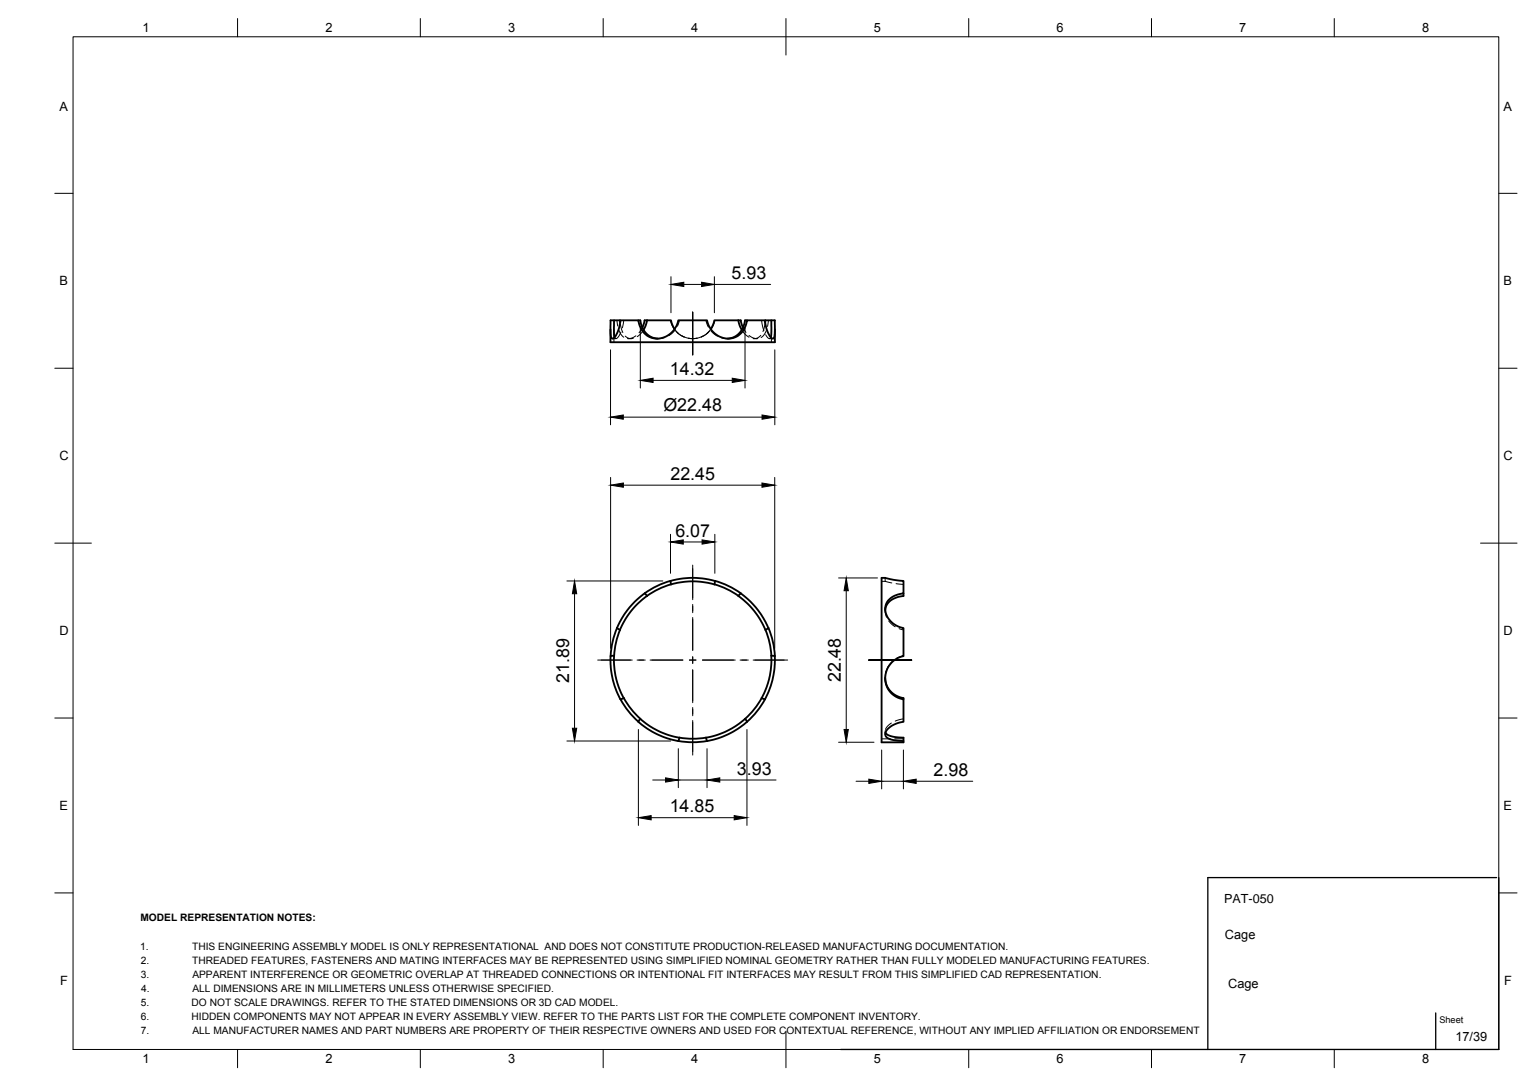
ISO-10303-21;
HEADER;
/* Generated by software containing ST-Developer
 * from STEP Tools, Inc. (www.steptools.com) 
 */

FILE_DESCRIPTION(
/* description */ ('Hand wheel with handle and shaft collar'),
/* implementation_level */ '2;1');

FILE_NAME(
/* name */ 'Cage.step',
/* time_stamp */ '2026-10-28T03:23:19-07:00',
/* author */ (''),
/* organization */ (''),
/* preprocessor_version */ 'ST-DEVELOPER v20.2',
/* originating_system */ 'Autodesk Translation Framework v15.17.0.0',
/* authorisation */ '');

FILE_SCHEMA (('AUTOMOTIVE_DESIGN { 1 0 10303 214 3 1 1 }'));
ENDSEC;

DATA;
#10=MECHANICAL_DESIGN_GEOMETRIC_PRESENTATION_REPRESENTATION('',(#413),#10510);
#227=B_SPLINE_CURVE_WITH_KNOTS('',3,(#8677,#8678,#8679,#8680,#8681,#8682,
#8683,#8684,#8685,#8686,#8687,#8688,#8689,#8690,#8691,#8692,#8693,#8694,
#8695,#8696,#8697,#8698),.UNSPECIFIED.,.F.,.F.,(4,2,2,2,2,2,2,2,2,2,4),
(0.0591825211272536,0.157966726598481,0.236950089897721,0.315933453196962,
0.391576304923761,0.46721915665056,0.54286200837736,0.618504860104159,0.697488223403399,
0.77647158670264,0.875255792173867),.UNSPECIFIED.);
#228=B_SPLINE_CURVE_WITH_KNOTS('',3,(#8702,#8703,#8704,#8705,#8706,#8707,
#8708,#8709,#8710,#8711,#8712,#8713,#8714,#8715,#8716,#8717,#8718,#8719,
#8720,#8721,#8722,#8723),.UNSPECIFIED.,.F.,.F.,(4,2,2,2,2,2,2,2,2,2,4),
(0.0581119756758434,0.106553146291161,0.213106292582322,0.30849933801665,
0.386091982889075,0.4636846277615,0.541277272633925,0.61886991750635,0.714262962940678,
0.820816109231839,0.869257279847157),.UNSPECIFIED.);
#229=B_SPLINE_CURVE_WITH_KNOTS('',3,(#8729,#8730,#8731,#8732,#8733,#8734,
#8735,#8736,#8737,#8738,#8739,#8740,#8741,#8742,#8743,#8744,#8745,#8746,
#8747,#8748,#8749,#8750),.UNSPECIFIED.,.F.,.F.,(4,2,2,2,2,2,2,2,2,2,4),
(0.0581119756758434,0.106553146291161,0.213106292582322,0.30849933801665,
0.386091982889075,0.4636846277615,0.541277272633925,0.61886991750635,0.714262962940679,
0.820816109231839,0.869257279847157),.UNSPECIFIED.);
#230=B_SPLINE_CURVE_WITH_KNOTS('',3,(#8754,#8755,#8756,#8757,#8758,#8759,
#8760,#8761,#8762,#8763,#8764,#8765,#8766,#8767,#8768,#8769,#8770,#8771,
#8772,#8773,#8774,#8775),.UNSPECIFIED.,.F.,.F.,(4,2,2,2,2,2,2,2,2,2,4),
(0.0581119756758433,0.106553146291161,0.213106292582322,0.308499338016649,
0.386091982889075,0.4636846277615,0.541277272633925,0.61886991750635,0.714262962940678,
0.820816109231839,0.869257279847157),.UNSPECIFIED.);
#231=B_SPLINE_CURVE_WITH_KNOTS('',3,(#8784,#8785,#8786,#8787,#8788,#8789,
#8790,#8791,#8792,#8793,#8794,#8795,#8796,#8797,#8798,#8799,#8800,#8801,
#8802,#8803,#8804,#8805),.UNSPECIFIED.,.F.,.F.,(4,2,2,2,2,2,2,2,2,2,4),
(0.0581119756758433,0.106553146291161,0.213106292582322,0.30849933801665,
0.386091982889075,0.4636846277615,0.541277272633925,0.61886991750635,0.714262962940678,
0.820816109231839,0.869257279847157),.UNSPECIFIED.);
#232=B_SPLINE_CURVE_WITH_KNOTS('',3,(#8809,#8810,#8811,#8812,#8813,#8814,
#8815,#8816,#8817,#8818,#8819,#8820,#8821,#8822,#8823,#8824,#8825,#8826,
#8827,#8828,#8829,#8830),.UNSPECIFIED.,.F.,.F.,(4,2,2,2,2,2,2,2,2,2,4),
(0.0581119756758434,0.106553146291161,0.213106292582322,0.30849933801665,
0.386091982889075,0.4636846277615,0.541277272633925,0.61886991750635,0.714262962940678,
0.820816109231839,0.869257279847157),.UNSPECIFIED.);
#233=B_SPLINE_CURVE_WITH_KNOTS('',3,(#8834,#8835,#8836,#8837,#8838,#8839,
#8840,#8841,#8842,#8843,#8844,#8845,#8846,#8847,#8848,#8849,#8850,#8851,
#8852,#8853,#8854,#8855),.UNSPECIFIED.,.F.,.F.,(4,2,2,2,2,2,2,2,2,2,4),
(0.0581119756758434,0.106553146291161,0.213106292582322,0.30849933801665,
0.386091982889075,0.4636846277615,0.541277272633925,0.61886991750635,0.714262962940678,
0.820816109231839,0.869257279847157),.UNSPECIFIED.);
#234=B_SPLINE_CURVE_WITH_KNOTS('',3,(#8859,#8860,#8861,#8862,#8863,#8864,
#8865,#8866,#8867,#8868,#8869,#8870,#8871,#8872,#8873,#8874,#8875,#8876,
#8877,#8878,#8879,#8880),.UNSPECIFIED.,.F.,.F.,(4,2,2,2,2,2,2,2,2,2,4),
(0.0581119756758433,0.106553146291161,0.213106292582322,0.30849933801665,
0.386091982889075,0.4636846277615,0.541277272633925,0.61886991750635,0.714262962940678,
0.820816109231839,0.869257279847157),.UNSPECIFIED.);
#235=B_SPLINE_CURVE_WITH_KNOTS('',3,(#8888,#8889,#8890,#8891,#8892,#8893,
#8894,#8895,#8896,#8897,#8898,#8899,#8900,#8901,#8902,#8903,#8904,#8905,
#8906,#8907,#8908,#8909),.UNSPECIFIED.,.F.,.F.,(4,2,2,2,2,2,2,2,2,2,4),
(0.0591825211272536,0.157966726598481,0.236950089897721,0.315933453196962,
0.391576304923761,0.467219156650561,0.54286200837736,0.618504860104159,
0.697488223403399,0.77647158670264,0.875255792173867),.UNSPECIFIED.);
#236=B_SPLINE_CURVE_WITH_KNOTS('',3,(#8917,#8918,#8919,#8920,#8921,#8922,
#8923,#8924,#8925,#8926,#8927,#8928,#8929,#8930,#8931,#8932,#8933,#8934,
#8935,#8936,#8937,#8938),.UNSPECIFIED.,.F.,.F.,(4,2,2,2,2,2,2,2,2,2,4),
(0.0591825211272536,0.157966726598481,0.236950089897722,0.315933453196962,
0.391576304923761,0.467219156650561,0.54286200837736,0.618504860104159,
0.697488223403399,0.77647158670264,0.875255792173867),.UNSPECIFIED.);
#237=B_SPLINE_CURVE_WITH_KNOTS('',3,(#8948,#8949,#8950,#8951,#8952,#8953,
#8954,#8955,#8956,#8957,#8958,#8959,#8960,#8961,#8962,#8963,#8964,#8965,
#8966,#8967,#8968,#8969),.UNSPECIFIED.,.F.,.F.,(4,2,2,2,2,2,2,2,2,2,4),
(0.0591825211272536,0.157966726598481,0.236950089897721,0.315933453196962,
0.391576304923761,0.46721915665056,0.54286200837736,0.618504860104159,0.697488223403399,
0.77647158670264,0.875255792173867),.UNSPECIFIED.);
#238=B_SPLINE_CURVE_WITH_KNOTS('',3,(#8977,#8978,#8979,#8980,#8981,#8982,
#8983,#8984,#8985,#8986,#8987,#8988,#8989,#8990,#8991,#8992,#8993,#8994,
#8995,#8996,#8997,#8998),.UNSPECIFIED.,.F.,.F.,(4,2,2,2,2,2,2,2,2,2,4),
(0.0591825211272536,0.157966726598481,0.236950089897721,0.315933453196962,
0.391576304923761,0.46721915665056,0.542862008377359,0.618504860104159,
0.697488223403399,0.776471586702639,0.875255792173867),.UNSPECIFIED.);
#239=B_SPLINE_CURVE_WITH_KNOTS('',3,(#9006,#9007,#9008,#9009,#9010,#9011,
#9012,#9013,#9014,#9015,#9016,#9017,#9018,#9019,#9020,#9021,#9022,#9023,
#9024,#9025,#9026,#9027),.UNSPECIFIED.,.F.,.F.,(4,2,2,2,2,2,2,2,2,2,4),
(0.0591825211272536,0.157966726598481,0.236950089897721,0.315933453196962,
0.391576304923761,0.46721915665056,0.54286200837736,0.618504860104159,0.697488223403399,
0.77647158670264,0.875255792173867),.UNSPECIFIED.);
#240=B_SPLINE_CURVE_WITH_KNOTS('',3,(#9036,#9037,#9038,#9039,#9040,#9041,
#9042,#9043,#9044,#9045,#9046,#9047,#9048,#9049,#9050,#9051,#9052,#9053,
#9054,#9055,#9056,#9057),.UNSPECIFIED.,.F.,.F.,(4,2,2,2,2,2,2,2,2,2,4),
(0.0591825211272536,0.157966726598481,0.236950089897721,0.315933453196962,
0.391576304923761,0.46721915665056,0.542862008377359,0.618504860104159,
0.697488223403399,0.776471586702639,0.875255792173867),.UNSPECIFIED.);
#274=SPHERICAL_SURFACE('',#5919,0.309556);
#275=SPHERICAL_SURFACE('',#5935,0.309556);
#276=SPHERICAL_SURFACE('',#5940,0.309556);
#277=SPHERICAL_SURFACE('',#5946,0.309556);
#278=SPHERICAL_SURFACE('',#5951,0.309556);
#279=SPHERICAL_SURFACE('',#5956,0.309556);
#280=SPHERICAL_SURFACE('',#5964,0.309556);
#343=SHAPE_REPRESENTATION_RELATIONSHIP('SRR','None',#10660,#375);
#375=ADVANCED_BREP_SHAPE_REPRESENTATION('',(#459),#10487);
#413=STYLED_ITEM('',(#10908),#459);
#459=MANIFOLD_SOLID_BREP('Continuous crown cage',#5313);
#543=FACE_BOUND('',#1263,.T.);
#651=PLANE('',#5932);
#652=PLANE('',#5937);
#653=PLANE('',#5942);
#654=PLANE('',#5948);
#655=PLANE('',#5953);
#656=PLANE('',#5962);
#657=PLANE('',#5966);
#658=PLANE('',#5967);
#871=FACE_OUTER_BOUND('',#1247,.T.);
#872=FACE_OUTER_BOUND('',#1248,.T.);
#873=FACE_OUTER_BOUND('',#1249,.T.);
#874=FACE_OUTER_BOUND('',#1250,.T.);
#875=FACE_OUTER_BOUND('',#1251,.T.);
#876=FACE_OUTER_BOUND('',#1252,.T.);
#877=FACE_OUTER_BOUND('',#1253,.T.);
#878=FACE_OUTER_BOUND('',#1254,.T.);
#879=FACE_OUTER_BOUND('',#1255,.T.);
#880=FACE_OUTER_BOUND('',#1256,.T.);
#881=FACE_OUTER_BOUND('',#1257,.T.);
#882=FACE_OUTER_BOUND('',#1258,.T.);
#883=FACE_OUTER_BOUND('',#1259,.T.);
#884=FACE_OUTER_BOUND('',#1260,.T.);
#885=FACE_OUTER_BOUND('',#1261,.T.);
#886=FACE_OUTER_BOUND('',#1262,.T.);
#887=FACE_OUTER_BOUND('',#1264,.T.);
#1247=EDGE_LOOP('',(#4001,#4002,#4003,#4004));
#1248=EDGE_LOOP('',(#4005,#4006,#4007,#4008,#4009,#4010,#4011,#4012,#4013,
#4014,#4015,#4016,#4017,#4018,#4019,#4020,#4021,#4022));
#1249=EDGE_LOOP('',(#4023,#4024,#4025,#4026));
#1250=EDGE_LOOP('',(#4027,#4028,#4029,#4030));
#1251=EDGE_LOOP('',(#4031,#4032,#4033,#4034));
#1252=EDGE_LOOP('',(#4035,#4036,#4037,#4038));
#1253=EDGE_LOOP('',(#4039,#4040,#4041,#4042,#4043,#4044));
#1254=EDGE_LOOP('',(#4045,#4046,#4047,#4048));
#1255=EDGE_LOOP('',(#4049,#4050,#4051,#4052));
#1256=EDGE_LOOP('',(#4053,#4054,#4055,#4056));
#1257=EDGE_LOOP('',(#4057,#4058,#4059,#4060));
#1258=EDGE_LOOP('',(#4061,#4062,#4063,#4064));
#1259=EDGE_LOOP('',(#4065,#4066,#4067,#4068,#4069,#4070,#4071,#4072,#4073,
#4074,#4075,#4076,#4077,#4078,#4079,#4080,#4081,#4082));
#1260=EDGE_LOOP('',(#4083,#4084,#4085,#4086));
#1261=EDGE_LOOP('',(#4087,#4088,#4089,#4090));
#1262=EDGE_LOOP('',(#4091));
#1263=EDGE_LOOP('',(#4092));
#1264=EDGE_LOOP('',(#4093,#4094,#4095,#4096));
#1637=LINE('',#8779,#1947);
#1638=LINE('',#9032,#1948);
#1947=VECTOR('',#7001,1.123812);
#1948=VECTOR('',#7070,1.076188);
#2231=CIRCLE('',#5920,0.303778037777585);
#2232=CIRCLE('',#5921,0.303778037777585);
#2233=CIRCLE('',#5923,1.123812);
#2234=CIRCLE('',#5924,1.123812);
#2235=CIRCLE('',#5925,1.123812);
#2236=CIRCLE('',#5926,1.123812);
#2237=CIRCLE('',#5927,1.123812);
#2238=CIRCLE('',#5928,1.123812);
#2239=CIRCLE('',#5929,1.123812);
#2240=CIRCLE('',#5930,1.123812);
#2241=CIRCLE('',#5931,1.123812);
#2242=CIRCLE('',#5933,1.076188);
#2243=CIRCLE('',#5934,0.303778037777585);
#2244=CIRCLE('',#5936,0.303778037777585);
#2245=CIRCLE('',#5938,1.076188);
#2246=CIRCLE('',#5939,0.303778037777585);
#2247=CIRCLE('',#5941,0.303778037777585);
#2248=CIRCLE('',#5943,1.076188);
#2249=CIRCLE('',#5944,1.076188);
#2250=CIRCLE('',#5945,0.303778037777585);
#2251=CIRCLE('',#5947,0.303778037777585);
#2252=CIRCLE('',#5949,1.076188);
#2253=CIRCLE('',#5950,0.303778037777585);
#2254=CIRCLE('',#5952,0.303778037777585);
#2255=CIRCLE('',#5954,1.076188);
#2256=CIRCLE('',#5955,0.303778037777585);
#2257=CIRCLE('',#5957,0.303778037777585);
#2258=CIRCLE('',#5959,1.076188);
#2259=CIRCLE('',#5960,1.076188);
#2260=CIRCLE('',#5961,1.076188);
#2261=CIRCLE('',#5963,0.303778037777585);
#2262=CIRCLE('',#5965,0.303778037777585);
#2599=VERTEX_POINT('',#8675);
#2600=VERTEX_POINT('',#8676);
#2601=VERTEX_POINT('',#8699);
#2602=VERTEX_POINT('',#8701);
#2603=VERTEX_POINT('',#8726);
#2604=VERTEX_POINT('',#8728);
#2605=VERTEX_POINT('',#8751);
#2606=VERTEX_POINT('',#8753);
#2607=VERTEX_POINT('',#8776);
#2608=VERTEX_POINT('',#8778);
#2609=VERTEX_POINT('',#8781);
#2610=VERTEX_POINT('',#8783);
#2611=VERTEX_POINT('',#8806);
#2612=VERTEX_POINT('',#8808);
#2613=VERTEX_POINT('',#8831);
#2614=VERTEX_POINT('',#8833);
#2615=VERTEX_POINT('',#8856);
#2616=VERTEX_POINT('',#8858);
#2617=VERTEX_POINT('',#8883);
#2618=VERTEX_POINT('',#8887);
#2619=VERTEX_POINT('',#8912);
#2620=VERTEX_POINT('',#8916);
#2621=VERTEX_POINT('',#8941);
#2622=VERTEX_POINT('',#8943);
#2623=VERTEX_POINT('',#8947);
#2624=VERTEX_POINT('',#8972);
#2625=VERTEX_POINT('',#8976);
#2626=VERTEX_POINT('',#9001);
#2627=VERTEX_POINT('',#9005);
#2628=VERTEX_POINT('',#9030);
#2629=VERTEX_POINT('',#9033);
#2630=VERTEX_POINT('',#9035);
#3118=EDGE_CURVE('',#2599,#2600,#227,.T.);
#3119=EDGE_CURVE('',#2601,#2599,#2231,.T.);
#3120=EDGE_CURVE('',#2602,#2601,#228,.T.);
#3121=EDGE_CURVE('',#2600,#2602,#2232,.T.);
#3122=EDGE_CURVE('',#2603,#2601,#2233,.T.);
#3123=EDGE_CURVE('',#2603,#2604,#229,.T.);
#3124=EDGE_CURVE('',#2605,#2604,#2234,.T.);
#3125=EDGE_CURVE('',#2605,#2606,#230,.T.);
#3126=EDGE_CURVE('',#2607,#2606,#2235,.T.);
#3127=EDGE_CURVE('',#2607,#2608,#1637,.T.);
#3128=EDGE_CURVE('',#2608,#2608,#2236,.T.);
#3129=EDGE_CURVE('',#2609,#2607,#2237,.T.);
#3130=EDGE_CURVE('',#2609,#2610,#231,.T.);
#3131=EDGE_CURVE('',#2611,#2610,#2238,.T.);
#3132=EDGE_CURVE('',#2611,#2612,#232,.T.);
#3133=EDGE_CURVE('',#2613,#2612,#2239,.T.);
#3134=EDGE_CURVE('',#2613,#2614,#233,.T.);
#3135=EDGE_CURVE('',#2615,#2614,#2240,.T.);
#3136=EDGE_CURVE('',#2615,#2616,#234,.T.);
#3137=EDGE_CURVE('',#2602,#2616,#2241,.T.);
#3138=EDGE_CURVE('',#2599,#2617,#2242,.T.);
#3139=EDGE_CURVE('',#2617,#2603,#2243,.T.);
#3140=EDGE_CURVE('',#2618,#2617,#235,.T.);
#3141=EDGE_CURVE('',#2604,#2618,#2244,.T.);
#3142=EDGE_CURVE('',#2618,#2619,#2245,.T.);
#3143=EDGE_CURVE('',#2619,#2605,#2246,.T.);
#3144=EDGE_CURVE('',#2620,#2619,#236,.T.);
#3145=EDGE_CURVE('',#2606,#2620,#2247,.T.);
#3146=EDGE_CURVE('',#2620,#2621,#2248,.T.);
#3147=EDGE_CURVE('',#2621,#2622,#2249,.T.);
#3148=EDGE_CURVE('',#2622,#2609,#2250,.T.);
#3149=EDGE_CURVE('',#2623,#2622,#237,.T.);
#3150=EDGE_CURVE('',#2610,#2623,#2251,.T.);
#3151=EDGE_CURVE('',#2623,#2624,#2252,.T.);
#3152=EDGE_CURVE('',#2624,#2611,#2253,.T.);
#3153=EDGE_CURVE('',#2625,#2624,#238,.T.);
#3154=EDGE_CURVE('',#2612,#2625,#2254,.T.);
#3155=EDGE_CURVE('',#2625,#2626,#2255,.T.);
#3156=EDGE_CURVE('',#2626,#2613,#2256,.T.);
#3157=EDGE_CURVE('',#2627,#2626,#239,.T.);
#3158=EDGE_CURVE('',#2614,#2627,#2257,.T.);
#3159=EDGE_CURVE('',#2628,#2628,#2258,.T.);
#3160=EDGE_CURVE('',#2628,#2621,#1638,.T.);
#3161=EDGE_CURVE('',#2629,#2600,#2259,.T.);
#3162=EDGE_CURVE('',#2629,#2630,#240,.T.);
#3163=EDGE_CURVE('',#2627,#2630,#2260,.T.);
#3164=EDGE_CURVE('',#2616,#2629,#2261,.T.);
#3165=EDGE_CURVE('',#2630,#2615,#2262,.T.);
#4001=ORIENTED_EDGE('',*,*,#3118,.F.);
#4002=ORIENTED_EDGE('',*,*,#3119,.F.);
#4003=ORIENTED_EDGE('',*,*,#3120,.F.);
#4004=ORIENTED_EDGE('',*,*,#3121,.F.);
#4005=ORIENTED_EDGE('',*,*,#3120,.T.);
#4006=ORIENTED_EDGE('',*,*,#3122,.F.);
#4007=ORIENTED_EDGE('',*,*,#3123,.T.);
#4008=ORIENTED_EDGE('',*,*,#3124,.F.);
#4009=ORIENTED_EDGE('',*,*,#3125,.T.);
#4010=ORIENTED_EDGE('',*,*,#3126,.F.);
#4011=ORIENTED_EDGE('',*,*,#3127,.T.);
#4012=ORIENTED_EDGE('',*,*,#3128,.F.);
#4013=ORIENTED_EDGE('',*,*,#3127,.F.);
#4014=ORIENTED_EDGE('',*,*,#3129,.F.);
#4015=ORIENTED_EDGE('',*,*,#3130,.T.);
#4016=ORIENTED_EDGE('',*,*,#3131,.F.);
#4017=ORIENTED_EDGE('',*,*,#3132,.T.);
#4018=ORIENTED_EDGE('',*,*,#3133,.F.);
#4019=ORIENTED_EDGE('',*,*,#3134,.T.);
#4020=ORIENTED_EDGE('',*,*,#3135,.F.);
#4021=ORIENTED_EDGE('',*,*,#3136,.T.);
#4022=ORIENTED_EDGE('',*,*,#3137,.F.);
#4023=ORIENTED_EDGE('',*,*,#3119,.T.);
#4024=ORIENTED_EDGE('',*,*,#3138,.T.);
#4025=ORIENTED_EDGE('',*,*,#3139,.T.);
#4026=ORIENTED_EDGE('',*,*,#3122,.T.);
#4027=ORIENTED_EDGE('',*,*,#3140,.F.);
#4028=ORIENTED_EDGE('',*,*,#3141,.F.);
#4029=ORIENTED_EDGE('',*,*,#3123,.F.);
#4030=ORIENTED_EDGE('',*,*,#3139,.F.);
#4031=ORIENTED_EDGE('',*,*,#3141,.T.);
#4032=ORIENTED_EDGE('',*,*,#3142,.T.);
#4033=ORIENTED_EDGE('',*,*,#3143,.T.);
#4034=ORIENTED_EDGE('',*,*,#3124,.T.);
#4035=ORIENTED_EDGE('',*,*,#3144,.F.);
#4036=ORIENTED_EDGE('',*,*,#3145,.F.);
#4037=ORIENTED_EDGE('',*,*,#3125,.F.);
#4038=ORIENTED_EDGE('',*,*,#3143,.F.);
#4039=ORIENTED_EDGE('',*,*,#3145,.T.);
#4040=ORIENTED_EDGE('',*,*,#3146,.T.);
#4041=ORIENTED_EDGE('',*,*,#3147,.T.);
#4042=ORIENTED_EDGE('',*,*,#3148,.T.);
#4043=ORIENTED_EDGE('',*,*,#3129,.T.);
#4044=ORIENTED_EDGE('',*,*,#3126,.T.);
#4045=ORIENTED_EDGE('',*,*,#3149,.F.);
#4046=ORIENTED_EDGE('',*,*,#3150,.F.);
#4047=ORIENTED_EDGE('',*,*,#3130,.F.);
#4048=ORIENTED_EDGE('',*,*,#3148,.F.);
#4049=ORIENTED_EDGE('',*,*,#3150,.T.);
#4050=ORIENTED_EDGE('',*,*,#3151,.T.);
#4051=ORIENTED_EDGE('',*,*,#3152,.T.);
#4052=ORIENTED_EDGE('',*,*,#3131,.T.);
#4053=ORIENTED_EDGE('',*,*,#3153,.F.);
#4054=ORIENTED_EDGE('',*,*,#3154,.F.);
#4055=ORIENTED_EDGE('',*,*,#3132,.F.);
#4056=ORIENTED_EDGE('',*,*,#3152,.F.);
#4057=ORIENTED_EDGE('',*,*,#3154,.T.);
#4058=ORIENTED_EDGE('',*,*,#3155,.T.);
#4059=ORIENTED_EDGE('',*,*,#3156,.T.);
#4060=ORIENTED_EDGE('',*,*,#3133,.T.);
#4061=ORIENTED_EDGE('',*,*,#3134,.F.);
#4062=ORIENTED_EDGE('',*,*,#3156,.F.);
#4063=ORIENTED_EDGE('',*,*,#3157,.F.);
#4064=ORIENTED_EDGE('',*,*,#3158,.F.);
#4065=ORIENTED_EDGE('',*,*,#3159,.F.);
#4066=ORIENTED_EDGE('',*,*,#3160,.T.);
#4067=ORIENTED_EDGE('',*,*,#3146,.F.);
#4068=ORIENTED_EDGE('',*,*,#3144,.T.);
#4069=ORIENTED_EDGE('',*,*,#3142,.F.);
#4070=ORIENTED_EDGE('',*,*,#3140,.T.);
#4071=ORIENTED_EDGE('',*,*,#3138,.F.);
#4072=ORIENTED_EDGE('',*,*,#3118,.T.);
#4073=ORIENTED_EDGE('',*,*,#3161,.F.);
#4074=ORIENTED_EDGE('',*,*,#3162,.T.);
#4075=ORIENTED_EDGE('',*,*,#3163,.F.);
#4076=ORIENTED_EDGE('',*,*,#3157,.T.);
#4077=ORIENTED_EDGE('',*,*,#3155,.F.);
#4078=ORIENTED_EDGE('',*,*,#3153,.T.);
#4079=ORIENTED_EDGE('',*,*,#3151,.F.);
#4080=ORIENTED_EDGE('',*,*,#3149,.T.);
#4081=ORIENTED_EDGE('',*,*,#3147,.F.);
#4082=ORIENTED_EDGE('',*,*,#3160,.F.);
#4083=ORIENTED_EDGE('',*,*,#3121,.T.);
#4084=ORIENTED_EDGE('',*,*,#3137,.T.);
#4085=ORIENTED_EDGE('',*,*,#3164,.T.);
#4086=ORIENTED_EDGE('',*,*,#3161,.T.);
#4087=ORIENTED_EDGE('',*,*,#3136,.F.);
#4088=ORIENTED_EDGE('',*,*,#3165,.F.);
#4089=ORIENTED_EDGE('',*,*,#3162,.F.);
#4090=ORIENTED_EDGE('',*,*,#3164,.F.);
#4091=ORIENTED_EDGE('',*,*,#3128,.T.);
#4092=ORIENTED_EDGE('',*,*,#3159,.T.);
#4093=ORIENTED_EDGE('',*,*,#3158,.T.);
#4094=ORIENTED_EDGE('',*,*,#3163,.T.);
#4095=ORIENTED_EDGE('',*,*,#3165,.T.);
#4096=ORIENTED_EDGE('',*,*,#3135,.T.);
#4918=CYLINDRICAL_SURFACE('',#5922,1.123812);
#4919=CYLINDRICAL_SURFACE('',#5958,1.076188);
#5083=ADVANCED_FACE('',(#871),#274,.F.);
#5084=ADVANCED_FACE('',(#872),#4918,.T.);
#5085=ADVANCED_FACE('',(#873),#651,.T.);
#5086=ADVANCED_FACE('',(#874),#275,.F.);
#5087=ADVANCED_FACE('',(#875),#652,.T.);
#5088=ADVANCED_FACE('',(#876),#276,.F.);
#5089=ADVANCED_FACE('',(#877),#653,.T.);
#5090=ADVANCED_FACE('',(#878),#277,.F.);
#5091=ADVANCED_FACE('',(#879),#654,.T.);
#5092=ADVANCED_FACE('',(#880),#278,.F.);
#5093=ADVANCED_FACE('',(#881),#655,.T.);
#5094=ADVANCED_FACE('',(#882),#279,.F.);
#5095=ADVANCED_FACE('',(#883),#4919,.F.);
#5096=ADVANCED_FACE('',(#884),#656,.T.);
#5097=ADVANCED_FACE('',(#885),#280,.F.);
#5098=ADVANCED_FACE('',(#886,#543),#657,.T.);
#5099=ADVANCED_FACE('',(#887),#658,.T.);
#5313=CLOSED_SHELL('',(#5083,#5084,#5085,#5086,#5087,#5088,#5089,#5090,
#5091,#5092,#5093,#5094,#5095,#5096,#5097,#5098,#5099));
#5918=AXIS2_PLACEMENT_3D('',#8673,#6985,#6986);
#5919=AXIS2_PLACEMENT_3D('',#8674,#6987,#6988);
#5920=AXIS2_PLACEMENT_3D('',#8700,#6989,#6990);
#5921=AXIS2_PLACEMENT_3D('',#8724,#6991,#6992);
#5922=AXIS2_PLACEMENT_3D('',#8725,#6993,#6994);
#5923=AXIS2_PLACEMENT_3D('',#8727,#6995,#6996);
#5924=AXIS2_PLACEMENT_3D('',#8752,#6997,#6998);
#5925=AXIS2_PLACEMENT_3D('',#8777,#6999,#7000);
#5926=AXIS2_PLACEMENT_3D('',#8780,#7002,#7003);
#5927=AXIS2_PLACEMENT_3D('',#8782,#7004,#7005);
#5928=AXIS2_PLACEMENT_3D('',#8807,#7006,#7007);
#5929=AXIS2_PLACEMENT_3D('',#8832,#7008,#7009);
#5930=AXIS2_PLACEMENT_3D('',#8857,#7010,#7011);
#5931=AXIS2_PLACEMENT_3D('',#8881,#7012,#7013);
#5932=AXIS2_PLACEMENT_3D('',#8882,#7014,#7015);
#5933=AXIS2_PLACEMENT_3D('',#8884,#7016,#7017);
#5934=AXIS2_PLACEMENT_3D('',#8885,#7018,#7019);
#5935=AXIS2_PLACEMENT_3D('',#8886,#7020,#7021);
#5936=AXIS2_PLACEMENT_3D('',#8910,#7022,#7023);
#5937=AXIS2_PLACEMENT_3D('',#8911,#7024,#7025);
#5938=AXIS2_PLACEMENT_3D('',#8913,#7026,#7027);
#5939=AXIS2_PLACEMENT_3D('',#8914,#7028,#7029);
#5940=AXIS2_PLACEMENT_3D('',#8915,#7030,#7031);
#5941=AXIS2_PLACEMENT_3D('',#8939,#7032,#7033);
#5942=AXIS2_PLACEMENT_3D('',#8940,#7034,#7035);
#5943=AXIS2_PLACEMENT_3D('',#8942,#7036,#7037);
#5944=AXIS2_PLACEMENT_3D('',#8944,#7038,#7039);
#5945=AXIS2_PLACEMENT_3D('',#8945,#7040,#7041);
#5946=AXIS2_PLACEMENT_3D('',#8946,#7042,#7043);
#5947=AXIS2_PLACEMENT_3D('',#8970,#7044,#7045);
#5948=AXIS2_PLACEMENT_3D('',#8971,#7046,#7047);
#5949=AXIS2_PLACEMENT_3D('',#8973,#7048,#7049);
#5950=AXIS2_PLACEMENT_3D('',#8974,#7050,#7051);
#5951=AXIS2_PLACEMENT_3D('',#8975,#7052,#7053);
#5952=AXIS2_PLACEMENT_3D('',#8999,#7054,#7055);
#5953=AXIS2_PLACEMENT_3D('',#9000,#7056,#7057);
#5954=AXIS2_PLACEMENT_3D('',#9002,#7058,#7059);
#5955=AXIS2_PLACEMENT_3D('',#9003,#7060,#7061);
#5956=AXIS2_PLACEMENT_3D('',#9004,#7062,#7063);
#5957=AXIS2_PLACEMENT_3D('',#9028,#7064,#7065);
#5958=AXIS2_PLACEMENT_3D('',#9029,#7066,#7067);
#5959=AXIS2_PLACEMENT_3D('',#9031,#7068,#7069);
#5960=AXIS2_PLACEMENT_3D('',#9034,#7071,#7072);
#5961=AXIS2_PLACEMENT_3D('',#9058,#7073,#7074);
#5962=AXIS2_PLACEMENT_3D('',#9059,#7075,#7076);
#5963=AXIS2_PLACEMENT_3D('',#9060,#7077,#7078);
#5964=AXIS2_PLACEMENT_3D('',#9061,#7079,#7080);
#5965=AXIS2_PLACEMENT_3D('',#9062,#7081,#7082);
#5966=AXIS2_PLACEMENT_3D('',#9063,#7083,#7084);
#5967=AXIS2_PLACEMENT_3D('',#9064,#7085,#7086);
#6985=DIRECTION('axis',(0.,0.,1.));
#6986=DIRECTION('refdir',(1.,0.,0.));
#6987=DIRECTION('center_axis',(0.,0.,1.));
#6988=DIRECTION('ref_axis',(1.,0.,0.));
#6989=DIRECTION('center_axis',(0.,-1.,0.));
#6990=DIRECTION('ref_axis',(0.,0.,-1.));
#6991=DIRECTION('center_axis',(0.,-1.,0.));
#6992=DIRECTION('ref_axis',(0.,0.,-1.));
#6993=DIRECTION('center_axis',(0.,1.,0.));
#6994=DIRECTION('ref_axis',(1.,0.,0.));
#6995=DIRECTION('center_axis',(0.,1.,0.));
#6996=DIRECTION('ref_axis',(1.,0.,0.));
#6997=DIRECTION('center_axis',(0.,1.,0.));
#6998=DIRECTION('ref_axis',(1.,0.,0.));
#6999=DIRECTION('center_axis',(0.,1.,0.));
#7000=DIRECTION('ref_axis',(1.,0.,0.));
#7001=DIRECTION('',(0.,-1.,0.));
#7002=DIRECTION('center_axis',(0.,-1.,0.));
#7003=DIRECTION('ref_axis',(1.,0.,0.));
#7004=DIRECTION('center_axis',(0.,1.,0.));
#7005=DIRECTION('ref_axis',(1.,0.,0.));
#7006=DIRECTION('center_axis',(0.,1.,0.));
#7007=DIRECTION('ref_axis',(1.,0.,0.));
#7008=DIRECTION('center_axis',(0.,1.,0.));
#7009=DIRECTION('ref_axis',(1.,0.,0.));
#7010=DIRECTION('center_axis',(0.,1.,0.));
#7011=DIRECTION('ref_axis',(1.,0.,0.));
#7012=DIRECTION('center_axis',(0.,1.,0.));
#7013=DIRECTION('ref_axis',(1.,0.,0.));
#7014=DIRECTION('center_axis',(0.,1.,0.));
#7015=DIRECTION('ref_axis',(1.,0.,0.));
#7016=DIRECTION('center_axis',(0.,-1.,0.));
#7017=DIRECTION('ref_axis',(1.,0.,0.));
#7018=DIRECTION('center_axis',(0.,-1.,0.));
#7019=DIRECTION('ref_axis',(0.,0.,-1.));
#7020=DIRECTION('center_axis',(8.96625347776458E-17,0.,1.));
#7021=DIRECTION('ref_axis',(1.,0.,0.));
#7022=DIRECTION('center_axis',(0.,-1.,0.));
#7023=DIRECTION('ref_axis',(0.,0.,-1.));
#7024=DIRECTION('center_axis',(0.,1.,0.));
#7025=DIRECTION('ref_axis',(1.,0.,0.));
#7026=DIRECTION('center_axis',(0.,-1.,0.));
#7027=DIRECTION('ref_axis',(1.,0.,0.));
#7028=DIRECTION('center_axis',(0.,-1.,0.));
#7029=DIRECTION('ref_axis',(0.,0.,-1.));
#7030=DIRECTION('center_axis',(0.,0.,1.));
#7031=DIRECTION('ref_axis',(1.,0.,0.));
#7032=DIRECTION('center_axis',(0.,-1.,0.));
#7033=DIRECTION('ref_axis',(0.,0.,-1.));
#7034=DIRECTION('center_axis',(0.,1.,0.));
#7035=DIRECTION('ref_axis',(1.,0.,0.));
#7036=DIRECTION('center_axis',(0.,-1.,0.));
#7037=DIRECTION('ref_axis',(1.,0.,0.));
#7038=DIRECTION('center_axis',(0.,-1.,0.));
#7039=DIRECTION('ref_axis',(1.,0.,0.));
#7040=DIRECTION('center_axis',(0.,-1.,0.));
#7041=DIRECTION('ref_axis',(0.,0.,-1.));
#7042=DIRECTION('center_axis',(0.,0.,1.));
#7043=DIRECTION('ref_axis',(1.,0.,0.));
#7044=DIRECTION('center_axis',(0.,-1.,0.));
#7045=DIRECTION('ref_axis',(0.,0.,-1.));
#7046=DIRECTION('center_axis',(0.,1.,0.));
#7047=DIRECTION('ref_axis',(1.,0.,0.));
#7048=DIRECTION('center_axis',(0.,-1.,0.));
#7049=DIRECTION('ref_axis',(1.,0.,0.));
#7050=DIRECTION('center_axis',(0.,-1.,0.));
#7051=DIRECTION('ref_axis',(0.,0.,-1.));
#7052=DIRECTION('center_axis',(8.96625347776458E-17,0.,1.));
#7053=DIRECTION('ref_axis',(1.,0.,0.));
#7054=DIRECTION('center_axis',(0.,-1.,0.));
#7055=DIRECTION('ref_axis',(0.,0.,-1.));
#7056=DIRECTION('center_axis',(0.,1.,0.));
#7057=DIRECTION('ref_axis',(1.,0.,0.));
#7058=DIRECTION('center_axis',(0.,-1.,0.));
#7059=DIRECTION('ref_axis',(1.,0.,0.));
#7060=DIRECTION('center_axis',(0.,-1.,0.));
#7061=DIRECTION('ref_axis',(0.,0.,-1.));
#7062=DIRECTION('center_axis',(0.,0.,1.));
#7063=DIRECTION('ref_axis',(1.,0.,0.));
#7064=DIRECTION('center_axis',(0.,-1.,0.));
#7065=DIRECTION('ref_axis',(0.,0.,-1.));
#7066=DIRECTION('center_axis',(0.,1.,0.));
#7067=DIRECTION('ref_axis',(1.,0.,0.));
#7068=DIRECTION('center_axis',(0.,1.,0.));
#7069=DIRECTION('ref_axis',(1.,0.,0.));
#7070=DIRECTION('',(0.,1.,0.));
#7071=DIRECTION('center_axis',(0.,-1.,0.));
#7072=DIRECTION('ref_axis',(1.,0.,0.));
#7073=DIRECTION('center_axis',(0.,-1.,0.));
#7074=DIRECTION('ref_axis',(1.,0.,0.));
#7075=DIRECTION('center_axis',(0.,1.,0.));
#7076=DIRECTION('ref_axis',(1.,0.,0.));
#7077=DIRECTION('center_axis',(0.,-1.,0.));
#7078=DIRECTION('ref_axis',(0.,0.,-1.));
#7079=DIRECTION('center_axis',(0.,0.,1.));
#7080=DIRECTION('ref_axis',(1.,0.,0.));
#7081=DIRECTION('center_axis',(0.,-1.,0.));
#7082=DIRECTION('ref_axis',(0.,0.,-1.));
#7083=DIRECTION('center_axis',(0.,-1.,0.));
#7084=DIRECTION('ref_axis',(-1.,0.,0.));
#7085=DIRECTION('center_axis',(0.,1.,0.));
#7086=DIRECTION('ref_axis',(1.,0.,0.));
#8673=CARTESIAN_POINT('',(0.,0.,0.));
#8674=CARTESIAN_POINT('Origin',(0.685838782044607,0.,0.860014630714833));
#8675=CARTESIAN_POINT('',(0.413083465285518,-0.05953,0.993751811093549));
#8676=CARTESIAN_POINT('',(0.876916659919095,-0.05953,0.623857181492959));
#8677=CARTESIAN_POINT('Ctrl Pts',(0.413083465285518,-0.05953,0.993751811093549));
#8678=CARTESIAN_POINT('Ctrl Pts',(0.419070565453383,-0.0925528133349865,
0.991263089003441));
#8679=CARTESIAN_POINT('Ctrl Pts',(0.430199341854858,-0.124911173756694,
0.986608710139579));
#8680=CARTESIAN_POINT('Ctrl Pts',(0.457978755888596,-0.177924977804098,
0.973971221090534));
#8681=CARTESIAN_POINT('Ctrl Pts',(0.473077587363685,-0.199697230012983,
0.966820759530997));
#8682=CARTESIAN_POINT('Ctrl Pts',(0.507057380724533,-0.237895043532788,
0.949440676105255));
#8683=CARTESIAN_POINT('Ctrl Pts',(0.525933334162555,-0.254319232363049,
0.939198248544428));
#8684=CARTESIAN_POINT('Ctrl Pts',(0.564362943424238,-0.28018331644634,0.916597376014514));
#8685=CARTESIAN_POINT('Ctrl Pts',(0.585840553788742,-0.29104845371857,0.903141581680914));
#8686=CARTESIAN_POINT('Ctrl Pts',(0.629305439856167,-0.30527573347708,0.873412008702649));
#8687=CARTESIAN_POINT('Ctrl Pts',(0.651278921914856,-0.308638795020976,
0.857118508332695));
#8688=CARTESIAN_POINT('Ctrl Pts',(0.690705563850638,-0.308638795020976,
0.825676810575914));
#8689=CARTESIAN_POINT('Ctrl Pts',(0.711480111898423,-0.30527573347708,0.807879894508811));
#8690=CARTESIAN_POINT('Ctrl Pts',(0.750136149454208,-0.29104845371857,0.772120216227122));
#8691=CARTESIAN_POINT('Ctrl Pts',(0.768033796848072,-0.28018331644634,0.754175290318038));
#8692=CARTESIAN_POINT('Ctrl Pts',(0.798619410861634,-0.254319232363049,
0.721738358858166));
#8693=CARTESIAN_POINT('Ctrl Pts',(0.812805334167529,-0.237895043532788,
0.705614819529209));
#8694=CARTESIAN_POINT('Ctrl Pts',(0.837310877969633,-0.199697230012983,
0.676354402927683));
#8695=CARTESIAN_POINT('Ctrl Pts',(0.847641868610495,-0.177924977804098,
0.663225258065736));
#8696=CARTESIAN_POINT('Ctrl Pts',(0.866144010579847,-0.124911173756694,
0.638954437806245));
#8697=CARTESIAN_POINT('Ctrl Pts',(0.873158080166742,-0.0925528133349865,
0.62914037979579));
#8698=CARTESIAN_POINT('Ctrl Pts',(0.876916659919095,-0.05953,0.623857181492959));
#8699=CARTESIAN_POINT('',(0.437601487681057,-0.05953,1.03511272300331));
#8700=CARTESIAN_POINT('Origin',(0.685838782044607,-0.05953,0.860014630714833));
#8701=CARTESIAN_POINT('',(0.911784794170997,-0.05953,0.656964154625313));
#8702=CARTESIAN_POINT('Ctrl Pts',(0.911784794170998,-0.0595300000000001,
0.656964154625312));
#8703=CARTESIAN_POINT('Ctrl Pts',(0.909827729890942,-0.0762225747374255,
0.659680317203144));
#8704=CARTESIAN_POINT('Ctrl Pts',(0.907004864562642,-0.0928409665394228,
0.663576540841106));
#8705=CARTESIAN_POINT('Ctrl Pts',(0.895234408667242,-0.144299303100741,
0.679480524217551));
#8706=CARTESIAN_POINT('Ctrl Pts',(0.882797231409153,-0.177024326825049,
0.695831250979106));
#8707=CARTESIAN_POINT('Ctrl Pts',(0.854332839576145,-0.227269801620064,
0.73042219438957));
#8708=CARTESIAN_POINT('Ctrl Pts',(0.834863020612702,-0.251265615809407,
0.752807465209441));
#8709=CARTESIAN_POINT('Ctrl Pts',(0.800439809856111,-0.279889827963178,
0.789147407129766));
#8710=CARTESIAN_POINT('Ctrl Pts',(0.781998747691871,-0.290879136862659,
0.80756613568454));
#8711=CARTESIAN_POINT('Ctrl Pts',(0.742239891936898,-0.305251990234487,
0.844254137480382));
#8712=CARTESIAN_POINT('Ctrl Pts',(0.720906778729541,-0.308638795020976,
0.862505527716294));
#8713=CARTESIAN_POINT('Ctrl Pts',(0.680463863683392,-0.308638795020976,
0.894757676234429));
#8714=CARTESIAN_POINT('Ctrl Pts',(0.657923009631182,-0.305251990234488,
0.91149460735272));
#8715=CARTESIAN_POINT('Ctrl Pts',(0.613307674922609,-0.290879136862659,
0.942092777160053));
#8716=CARTESIAN_POINT('Ctrl Pts',(0.591247219971725,-0.279889827963178,
0.955972930713954));
#8717=CARTESIAN_POINT('Ctrl Pts',(0.548158511259202,-0.251265615809407,
0.981446681891443));
#8718=CARTESIAN_POINT('Ctrl Pts',(0.522002043615455,-0.227269801620063,
0.995447160474328));
#8719=CARTESIAN_POINT('Ctrl Pts',(0.481944444320713,-0.177024326825049,
1.01550068154148));
#8720=CARTESIAN_POINT('Ctrl Pts',(0.463236132117164,-0.14429930310074,1.0239876538093));
#8721=CARTESIAN_POINT('Ctrl Pts',(0.445111721969657,-0.0928409665394226,
1.03192403056628));
#8722=CARTESIAN_POINT('Ctrl Pts',(0.440685038163619,-0.0762225747374254,
1.03380912944435));
#8723=CARTESIAN_POINT('Ctrl Pts',(0.437601487681056,-0.05953,1.03511272300331));
#8724=CARTESIAN_POINT('Origin',(0.685838782044607,-0.05953,0.860014630714833));
#8725=CARTESIAN_POINT('Origin',(0.,-0.208355,0.));
#8726=CARTESIAN_POINT('',(0.0548532617164168,-0.05953,1.12247250791415));
#8727=CARTESIAN_POINT('Origin',(0.,-0.05953,0.));
#8728=CARTESIAN_POINT('',(-0.536443649899848,-0.05953,0.987512846410683));
#8729=CARTESIAN_POINT('Ctrl Pts',(0.0548532617164173,-0.0595300000000001,
1.12247250791414));
#8730=CARTESIAN_POINT('Ctrl Pts',(0.05150947068137,-0.0762225747374254,
1.12263591311425));
#8731=CARTESIAN_POINT('Ctrl Pts',(0.0467032526342597,-0.0928409665394227,
1.12285816383385));
#8732=CARTESIAN_POINT('Ctrl Pts',(0.0269302585198975,-0.144299303100741,
1.12357162229597));
#8733=CARTESIAN_POINT('Ctrl Pts',(0.006392292392153,-0.177024326825049,
1.12404235695137));
#8734=CARTESIAN_POINT('Ctrl Pts',(-0.0383992541984087,-0.227269801620063,
1.12335509974011));
#8735=CARTESIAN_POINT('Ctrl Pts',(-0.0680399972366993,-0.251265615809407,
1.12208997038458));
#8736=CARTESIAN_POINT('Ctrl Pts',(-0.117914228755037,-0.279889827963178,
1.1178344036749));
#8737=CARTESIAN_POINT('Ctrl Pts',(-0.14381238480104,-0.290879136862659,
1.11490049012186));
#8738=CARTESIAN_POINT('Ctrl Pts',(-0.19728546073067,-0.305251990234488,
1.10669035995599));
#8739=CARTESIAN_POINT('Ctrl Pts',(-0.224855950742601,-0.308638795020976,
1.10139101611326));
#8740=CARTESIAN_POINT('Ctrl Pts',(-0.275287440920027,-0.308638795020976,
1.0898803575765));
#8741=CARTESIAN_POINT('Ctrl Pts',(-0.302426893214945,-0.305251990234488,
1.08269251410343));
#8742=CARTESIAN_POINT('Ctrl Pts',(-0.35416671187353,-0.290879136862659,
1.06688848765783));
#8743=CARTESIAN_POINT('Ctrl Pts',(-0.3787731215897,-0.279889827963178,1.05829506364875));
#8744=CARTESIAN_POINT('Ctrl Pts',(-0.425554672694338,-0.251265615809407,
1.04048957871266));
#8745=CARTESIAN_POINT('Ctrl Pts',(-0.452808978448581,-0.227269801620063,
1.02876878445619));
#8746=CARTESIAN_POINT('Ctrl Pts',(-0.493462957200432,-0.177024326825049,
1.0099536580922));
#8747=CARTESIAN_POINT('Ctrl Pts',(-0.511762781179148,-0.14429930310074,
1.00061845128527));
#8748=CARTESIAN_POINT('Ctrl Pts',(-0.529268075276157,-0.0928409665394226,
0.991396466802468));
#8749=CARTESIAN_POINT('Ctrl Pts',(-0.533501897135713,-0.0762225747374254,
0.989110885965947));
#8750=CARTESIAN_POINT('Ctrl Pts',(-0.536443649899848,-0.0595300000000001,
0.987512846410683));
#8751=CARTESIAN_POINT('',(-0.843383895613249,-0.05953,0.742736168477219));
#8752=CARTESIAN_POINT('Origin',(0.,-0.05953,0.));
#8753=CARTESIAN_POINT('',(-1.10653577764992,-0.05953,0.196295654879792));
#8754=CARTESIAN_POINT('Ctrl Pts',(-0.843383895613249,-0.0595300000000001,
0.742736168477219));
#8755=CARTESIAN_POINT('Ctrl Pts',(-0.84559647055299,-0.0762225747374255,
0.740223768851062));
#8756=CARTESIAN_POINT('Ctrl Pts',(-0.848766861100456,-0.0928409665394227,
0.736604687327351));
#8757=CARTESIAN_POINT('Ctrl Pts',(-0.861652925570091,-0.144299303100741,
0.721590372101268));
#8758=CARTESIAN_POINT('Ctrl Pts',(-0.87482617317514,-0.177024326825049,
0.705826641853758));
#8759=CARTESIAN_POINT('Ctrl Pts',(-0.902215926359523,-0.227269801620063,
0.670378702718353));
#8760=CARTESIAN_POINT('Ctrl Pts',(-0.919707509403859,-0.251265615809407,
0.646415841396062));
#8761=CARTESIAN_POINT('Ctrl Pts',(-0.947476448101718,-0.279889827963178,
0.604769294586516));
#8762=CARTESIAN_POINT('Ctrl Pts',(-0.961329858300736,-0.290879136862659,
0.582692035672022));
#8763=CARTESIAN_POINT('Ctrl Pts',(-0.988250837578047,-0.305251990234488,
0.535766169015486));
#8764=CARTESIAN_POINT('Ctrl Pts',(-1.00129756308006,-0.308638795020976,
0.510906605094603));
#8765=CARTESIAN_POINT('Ctrl Pts',(-1.02374168767024,-0.308638795020976,
0.46430090015576));
#8766=CARTESIAN_POINT('Ctrl Pts',(-1.03504317708586,-0.305251990234488,
0.438600874831839));
#8767=CARTESIAN_POINT('Ctrl Pts',(-1.05494634094458,-0.290879136862659,
0.388295406390235));
#8768=CARTESIAN_POINT('Ctrl Pts',(-1.06356957703048,-0.279889827963178,
0.363699428370917));
#8769=CARTESIAN_POINT('Ctrl Pts',(-1.0788165083757,-0.251265615809407,0.316022600643821));
#8770=CARTESIAN_POINT('Ctrl Pts',(-1.08664560412098,-0.227269801620063,
0.287406530683752));
#8771=CARTESIAN_POINT('Ctrl Pts',(-1.09728268713976,-0.177024326825049,
0.243890930799337));
#8772=CARTESIAN_POINT('Ctrl Pts',(-1.10139388218929,-0.144299303100741,
0.22376314604679));
#8773=CARTESIAN_POINT('Ctrl Pts',(-1.10509821673782,-0.0928409665394227,
0.204327142733961));
#8774=CARTESIAN_POINT('Ctrl Pts',(-1.10595102243643,-0.0762225747374254,
0.199591971170104));
#8775=CARTESIAN_POINT('Ctrl Pts',(-1.10653577764992,-0.0595300000000001,
0.196295654879792));
#8776=CARTESIAN_POINT('',(-1.123812,-0.05953,1.37627276864339E-16));
#8777=CARTESIAN_POINT('Origin',(0.,-0.05953,0.));
#8778=CARTESIAN_POINT('',(-1.123812,-0.35718,1.37627276864339E-16));
#8779=CARTESIAN_POINT('',(-1.123812,-0.208355,1.37627276864339E-16));
#8780=CARTESIAN_POINT('Origin',(0.,-0.35718,0.));
#8781=CARTESIAN_POINT('',(-1.10653577764992,-0.05953,-0.196295654879793));
#8782=CARTESIAN_POINT('Origin',(0.,-0.05953,0.));
#8783=CARTESIAN_POINT('',(-0.843383895613249,-0.05953,-0.742736168477219));
#8784=CARTESIAN_POINT('Ctrl Pts',(-1.10653577764992,-0.0595300000000001,
-0.196295654879792));
#8785=CARTESIAN_POINT('Ctrl Pts',(-1.10595102243643,-0.0762225747374255,
-0.199591971170104));
#8786=CARTESIAN_POINT('Ctrl Pts',(-1.10509821673782,-0.0928409665394228,
-0.204327142733962));
#8787=CARTESIAN_POINT('Ctrl Pts',(-1.10139388218929,-0.144299303100741,
-0.22376314604679));
#8788=CARTESIAN_POINT('Ctrl Pts',(-1.09728268713976,-0.177024326825049,
-0.243890930799338));
#8789=CARTESIAN_POINT('Ctrl Pts',(-1.08664560412098,-0.227269801620063,
-0.287406530683753));
#8790=CARTESIAN_POINT('Ctrl Pts',(-1.0788165083757,-0.251265615809407,-0.316022600643821));
#8791=CARTESIAN_POINT('Ctrl Pts',(-1.06356957703048,-0.279889827963178,
-0.363699428370918));
#8792=CARTESIAN_POINT('Ctrl Pts',(-1.05494634094458,-0.290879136862659,
-0.388295406390235));
#8793=CARTESIAN_POINT('Ctrl Pts',(-1.03504317708586,-0.305251990234488,
-0.438600874831839));
#8794=CARTESIAN_POINT('Ctrl Pts',(-1.02374168767024,-0.308638795020976,
-0.46430090015576));
#8795=CARTESIAN_POINT('Ctrl Pts',(-1.00129756308006,-0.308638795020976,
-0.510906605094603));
#8796=CARTESIAN_POINT('Ctrl Pts',(-0.988250837578047,-0.305251990234488,
-0.535766169015486));
#8797=CARTESIAN_POINT('Ctrl Pts',(-0.961329858300736,-0.290879136862659,
-0.582692035672022));
#8798=CARTESIAN_POINT('Ctrl Pts',(-0.947476448101718,-0.279889827963178,
-0.604769294586516));
#8799=CARTESIAN_POINT('Ctrl Pts',(-0.919707509403859,-0.251265615809407,
-0.646415841396062));
#8800=CARTESIAN_POINT('Ctrl Pts',(-0.902215926359523,-0.227269801620064,
-0.670378702718353));
#8801=CARTESIAN_POINT('Ctrl Pts',(-0.87482617317514,-0.177024326825049,
-0.705826641853758));
#8802=CARTESIAN_POINT('Ctrl Pts',(-0.861652925570091,-0.144299303100741,
-0.721590372101268));
#8803=CARTESIAN_POINT('Ctrl Pts',(-0.848766861100456,-0.0928409665394229,
-0.736604687327351));
#8804=CARTESIAN_POINT('Ctrl Pts',(-0.84559647055299,-0.0762225747374255,
-0.740223768851063));
#8805=CARTESIAN_POINT('Ctrl Pts',(-0.843383895613249,-0.0595300000000001,
-0.742736168477219));
#8806=CARTESIAN_POINT('',(-0.536443649899847,-0.05953,-0.987512846410683));
#8807=CARTESIAN_POINT('Origin',(0.,-0.05953,0.));
#8808=CARTESIAN_POINT('',(0.0548532617164172,-0.05953,-1.12247250791415));
#8809=CARTESIAN_POINT('Ctrl Pts',(-0.536443649899848,-0.0595300000000001,
-0.987512846410683));
#8810=CARTESIAN_POINT('Ctrl Pts',(-0.533501897135712,-0.0762225747374254,
-0.989110885965947));
#8811=CARTESIAN_POINT('Ctrl Pts',(-0.529268075276156,-0.0928409665394227,
-0.991396466802469));
#8812=CARTESIAN_POINT('Ctrl Pts',(-0.511762781179147,-0.144299303100741,
-1.00061845128527));
#8813=CARTESIAN_POINT('Ctrl Pts',(-0.493462957200432,-0.177024326825049,
-1.0099536580922));
#8814=CARTESIAN_POINT('Ctrl Pts',(-0.45280897844858,-0.227269801620063,
-1.02876878445619));
#8815=CARTESIAN_POINT('Ctrl Pts',(-0.425554672694337,-0.251265615809407,
-1.04048957871266));
#8816=CARTESIAN_POINT('Ctrl Pts',(-0.3787731215897,-0.279889827963178,-1.05829506364875));
#8817=CARTESIAN_POINT('Ctrl Pts',(-0.354166711873529,-0.290879136862659,
-1.06688848765783));
#8818=CARTESIAN_POINT('Ctrl Pts',(-0.302426893214944,-0.305251990234488,
-1.08269251410343));
#8819=CARTESIAN_POINT('Ctrl Pts',(-0.275287440920027,-0.308638795020976,
-1.0898803575765));
#8820=CARTESIAN_POINT('Ctrl Pts',(-0.224855950742601,-0.308638795020976,
-1.10139101611326));
#8821=CARTESIAN_POINT('Ctrl Pts',(-0.19728546073067,-0.305251990234488,
-1.10669035995599));
#8822=CARTESIAN_POINT('Ctrl Pts',(-0.143812384801039,-0.290879136862659,
-1.11490049012186));
#8823=CARTESIAN_POINT('Ctrl Pts',(-0.117914228755037,-0.279889827963178,
-1.1178344036749));
#8824=CARTESIAN_POINT('Ctrl Pts',(-0.0680399972366989,-0.251265615809407,
-1.12208997038458));
#8825=CARTESIAN_POINT('Ctrl Pts',(-0.0383992541984084,-0.227269801620063,
-1.12335509974011));
#8826=CARTESIAN_POINT('Ctrl Pts',(0.00639229239215326,-0.177024326825049,
-1.12404235695137));
#8827=CARTESIAN_POINT('Ctrl Pts',(0.0269302585198977,-0.144299303100741,
-1.12357162229597));
#8828=CARTESIAN_POINT('Ctrl Pts',(0.04670325263426,-0.0928409665394228,
-1.12285816383385));
#8829=CARTESIAN_POINT('Ctrl Pts',(0.0515094706813703,-0.0762225747374255,
-1.12263591311425));
#8830=CARTESIAN_POINT('Ctrl Pts',(0.0548532617164176,-0.0595300000000001,
-1.12247250791414));
#8831=CARTESIAN_POINT('',(0.437601487681057,-0.05953,-1.03511272300331));
#8832=CARTESIAN_POINT('Origin',(0.,-0.05953,0.));
#8833=CARTESIAN_POINT('',(0.911784794170997,-0.05953,-0.656964154625313));
#8834=CARTESIAN_POINT('Ctrl Pts',(0.437601487681056,-0.0595300000000001,
-1.03511272300331));
#8835=CARTESIAN_POINT('Ctrl Pts',(0.440685038163619,-0.0762225747374255,
-1.03380912944435));
#8836=CARTESIAN_POINT('Ctrl Pts',(0.445111721969657,-0.0928409665394228,
-1.03192403056628));
#8837=CARTESIAN_POINT('Ctrl Pts',(0.463236132117164,-0.144299303100741,
-1.0239876538093));
#8838=CARTESIAN_POINT('Ctrl Pts',(0.481944444320713,-0.177024326825049,
-1.01550068154148));
#8839=CARTESIAN_POINT('Ctrl Pts',(0.522002043615455,-0.227269801620064,
-0.995447160474328));
#8840=CARTESIAN_POINT('Ctrl Pts',(0.548158511259203,-0.251265615809407,
-0.981446681891443));
#8841=CARTESIAN_POINT('Ctrl Pts',(0.591247219971725,-0.279889827963178,
-0.955972930713954));
#8842=CARTESIAN_POINT('Ctrl Pts',(0.613307674922609,-0.290879136862659,
-0.942092777160053));
#8843=CARTESIAN_POINT('Ctrl Pts',(0.657923009631182,-0.305251990234487,
-0.91149460735272));
#8844=CARTESIAN_POINT('Ctrl Pts',(0.680463863683393,-0.308638795020976,
-0.894757676234429));
#8845=CARTESIAN_POINT('Ctrl Pts',(0.720906778729542,-0.308638795020976,
-0.862505527716294));
#8846=CARTESIAN_POINT('Ctrl Pts',(0.742239891936899,-0.305251990234488,
-0.844254137480381));
#8847=CARTESIAN_POINT('Ctrl Pts',(0.781998747691872,-0.290879136862659,
-0.80756613568454));
#8848=CARTESIAN_POINT('Ctrl Pts',(0.800439809856112,-0.279889827963178,
-0.789147407129765));
#8849=CARTESIAN_POINT('Ctrl Pts',(0.834863020612702,-0.251265615809407,
-0.752807465209441));
#8850=CARTESIAN_POINT('Ctrl Pts',(0.854332839576145,-0.227269801620064,
-0.73042219438957));
#8851=CARTESIAN_POINT('Ctrl Pts',(0.882797231409153,-0.177024326825049,
-0.695831250979106));
#8852=CARTESIAN_POINT('Ctrl Pts',(0.895234408667242,-0.144299303100741,
-0.679480524217551));
#8853=CARTESIAN_POINT('Ctrl Pts',(0.907004864562642,-0.0928409665394228,
-0.663576540841106));
#8854=CARTESIAN_POINT('Ctrl Pts',(0.909827729890942,-0.0762225747374256,
-0.659680317203144));
#8855=CARTESIAN_POINT('Ctrl Pts',(0.911784794170998,-0.0595300000000001,
-0.656964154625312));
#8856=CARTESIAN_POINT('',(1.08212377959455,-0.05953,-0.303251606722892));
#8857=CARTESIAN_POINT('Origin',(0.,-0.05953,0.));
#8858=CARTESIAN_POINT('',(1.08212377959455,-0.05953,0.303251606722892));
#8859=CARTESIAN_POINT('Ctrl Pts',(1.08212377959455,-0.0595300000000001,
-0.303251606722892));
#8860=CARTESIAN_POINT('Ctrl Pts',(1.0830271513892,-0.0762225747374255,-0.300028012588062));
#8861=CARTESIAN_POINT('Ctrl Pts',(1.08431331394788,-0.0928409665394228,
-0.2953917518996));
#8862=CARTESIAN_POINT('Ctrl Pts',(1.08940878963422,-0.144299303100741,-0.276273267473431));
#8863=CARTESIAN_POINT('Ctrl Pts',(1.09443784939331,-0.177024326825049,-0.256354979351213));
#8864=CARTESIAN_POINT('Ctrl Pts',(1.10373487993589,-0.227269801620064,-0.212533521233765));
#8865=CARTESIAN_POINT('Ctrl Pts',(1.10909715583869,-0.251265615809407,-0.183354415742157));
#8866=CARTESIAN_POINT('Ctrl Pts',(1.1160463456491,-0.279889827963178,-0.133783682657561));
#8867=CARTESIAN_POINT('Ctrl Pts',(1.11894887330541,-0.290879136862659,-0.107881990270302));
#8868=CARTESIAN_POINT('Ctrl Pts',(1.12284346704144,-0.305251990234488,-0.0539226701638766));
#8869=CARTESIAN_POINT('Ctrl Pts',(1.123812,-0.308638795020976,-0.025864214957475));
#8870=CARTESIAN_POINT('Ctrl Pts',(1.123812,-0.308638795020976,0.025864214957475));
#8871=CARTESIAN_POINT('Ctrl Pts',(1.12284346704144,-0.305251990234488,0.0539226701638766));
#8872=CARTESIAN_POINT('Ctrl Pts',(1.11894887330541,-0.290879136862659,0.107881990270302));
#8873=CARTESIAN_POINT('Ctrl Pts',(1.1160463456491,-0.279889827963178,0.133783682657561));
#8874=CARTESIAN_POINT('Ctrl Pts',(1.10909715583869,-0.251265615809407,0.183354415742157));
#8875=CARTESIAN_POINT('Ctrl Pts',(1.10373487993589,-0.227269801620064,0.212533521233765));
#8876=CARTESIAN_POINT('Ctrl Pts',(1.09443784939331,-0.177024326825049,0.256354979351213));
#8877=CARTESIAN_POINT('Ctrl Pts',(1.08940878963422,-0.144299303100741,0.276273267473431));
#8878=CARTESIAN_POINT('Ctrl Pts',(1.08431331394788,-0.0928409665394228,
0.2953917518996));
#8879=CARTESIAN_POINT('Ctrl Pts',(1.0830271513892,-0.0762225747374255,0.300028012588062));
#8880=CARTESIAN_POINT('Ctrl Pts',(1.08212377959455,-0.0595300000000001,
0.303251606722892));
#8881=CARTESIAN_POINT('Origin',(0.,-0.05953,0.));
#8882=CARTESIAN_POINT('Origin',(0.,-0.05953,0.));
#8883=CARTESIAN_POINT('',(0.0589974094846122,-0.05953,1.07456964270265));
#8884=CARTESIAN_POINT('Origin',(0.,-0.05953,0.));
#8885=CARTESIAN_POINT('Origin',(-0.244773027351946,-0.05953,1.07242070340001));
#8886=CARTESIAN_POINT('Origin',(-0.244773027351946,0.,1.07242070340001));
#8887=CARTESIAN_POINT('',(-0.519393123750572,-0.05953,0.942555777842682));
#8888=CARTESIAN_POINT('Ctrl Pts',(-0.519393123750572,-0.05953,0.942555777842682));
#8889=CARTESIAN_POINT('Ctrl Pts',(-0.513714466572041,-0.0925528133349865,
0.945684988399766));
#8890=CARTESIAN_POINT('Ctrl Pts',(-0.503136848051455,-0.124911173756694,
0.951483858396181));
#8891=CARTESIAN_POINT('Ctrl Pts',(-0.47593627990192,-0.177924977804098,
0.965323333309091));
#8892=CARTESIAN_POINT('Ctrl Pts',(-0.460931856495794,-0.199697230012983,
0.972669835243841));
#8893=CARTESIAN_POINT('Ctrl Pts',(-0.426157505475872,-0.237895043532788,
0.988400002689705));
#8894=CARTESIAN_POINT('Ctrl Pts',(-0.406380688682952,-0.254319232363049,
0.996771768218699));
#8895=CARTESIAN_POINT('Ctrl Pts',(-0.364750145543744,-0.28018331644634,
1.01272583306292));
#8896=CARTESIAN_POINT('Ctrl Pts',(-0.340838910881557,-0.29104845371857,
1.02112815447116));
#8897=CARTESIAN_POINT('Ctrl Pts',(-0.290495481564827,-0.30527573347708,
1.036574285215));
#8898=CARTESIAN_POINT('Ctrl Pts',(-0.264056468041074,-0.308638795020976,
1.04359501395068));
#8899=CARTESIAN_POINT('Ctrl Pts',(-0.214892249704082,-0.308638795020976,
1.05481642595959));
#8900=CARTESIAN_POINT('Ctrl Pts',(-0.188025341585962,-0.30527573347708,
1.05996242598502));
#8901=CARTESIAN_POINT('Ctrl Pts',(-0.135965654106109,-0.29104845371857,
1.06788913840721));
#8902=CARTESIAN_POINT('Ctrl Pts',(-0.110776745452494,-0.28018331644634,
1.07069360430242));
#8903=CARTESIAN_POINT('Ctrl Pts',(-0.0663467128214646,-0.254319232363049,
1.07438230428002));
#8904=CARTESIAN_POINT('Ctrl Pts',(-0.0448960436540983,-0.237895043532788,
1.07542044338697));
#8905=CARTESIAN_POINT('Ctrl Pts',(-0.00674037211528124,-0.199697230012983,
1.07633607767727));
#8906=CARTESIAN_POINT('Ctrl Pts',(0.00996567398334777,-0.177924977804098,
1.07622728347683));
#8907=CARTESIAN_POINT('Ctrl Pts',(0.0404772621979741,-0.124911173756694,
1.07556023164702));
#8908=CARTESIAN_POINT('Ctrl Pts',(0.0525234025782719,-0.0925528133349865,
1.07492508698591));
#8909=CARTESIAN_POINT('Ctrl Pts',(0.0589974094846124,-0.05953,1.07456964270265));
#8910=CARTESIAN_POINT('Origin',(-0.244773027351946,-0.05953,1.07242070340001));
#8911=CARTESIAN_POINT('Origin',(0.,-0.05953,0.));
#8912=CARTESIAN_POINT('',(-0.803348093619616,-0.05953,0.716109245731214));
#8913=CARTESIAN_POINT('Origin',(0.,-0.05953,0.));
#8914=CARTESIAN_POINT('Origin',(-0.991065754692661,-0.05953,0.477272113029314));
#8915=CARTESIAN_POINT('Origin',(-0.991065754692661,0.,0.477272113029314));
#8916=CARTESIAN_POINT('',(-1.06075609691358,-0.05953,0.181596019242328));
#8917=CARTESIAN_POINT('Ctrl Pts',(-1.06075609691358,-0.05953,0.181596019242328));
#8918=CARTESIAN_POINT('Ctrl Pts',(-1.05966202740332,-0.0925528133349865,
0.187986803072856));
#8919=CARTESIAN_POINT('Ctrl Pts',(-1.05760072925372,-0.124911173756694,
0.199872254546857));
#8920=CARTESIAN_POINT('Ctrl Pts',(-1.05146158959546,-0.177924977804098,
0.22976728653846));
#8921=CARTESIAN_POINT('Ctrl Pts',(-1.04785021111757,-0.199697230012983,
0.246078686169301));
#8922=CARTESIAN_POINT('Ctrl Pts',(-1.03846709802406,-0.237895043532788,
0.283073967563097));
#8923=CARTESIAN_POINT('Ctrl Pts',(-1.03268176429485,-0.254319232363049,
0.303755815985685));
#8924=CARTESIAN_POINT('Ctrl Pts',(-1.01919893537026,-0.28018331644634,0.346251081972725));
#8925=CARTESIAN_POINT('Ctrl Pts',(-1.01085972381132,-0.29104845371857,0.370184399726282));
#8926=CARTESIAN_POINT('Ctrl Pts',(-0.99154738033959,-0.30527573347708,0.419174982698463));
#8927=CARTESIAN_POINT('Ctrl Pts',(-0.980551951791748,-0.308638795020976,
0.444223188605045));
#8928=CARTESIAN_POINT('Ctrl Pts',(-0.958671816228589,-0.308638795020976,
0.489657758261848));
#8929=CARTESIAN_POINT('Ctrl Pts',(-0.945943877838127,-0.30527573347708,
0.51387163140139));
#8930=CARTESIAN_POINT('Ctrl Pts',(-0.91968254693063,-0.29104845371857,0.559515758398093));
#8931=CARTESIAN_POINT('Ctrl Pts',(-0.906170138993533,-0.28018331644634,
0.580957796077825));
#8932=CARTESIAN_POINT('Ctrl Pts',(-0.8813524085237,-0.254319232363049,0.617994461173994));
#8933=CARTESIAN_POINT('Ctrl Pts',(-0.868789784891799,-0.237895043532788,
0.635412538795143));
#8934=CARTESIAN_POINT('Ctrl Pts',(-0.845715984518854,-0.199697230012983,
0.66581473268113));
#8935=CARTESIAN_POINT('Ctrl Pts',(-0.835214876415962,-0.177924977804098,
0.678808213394124));
#8936=CARTESIAN_POINT('Ctrl Pts',(-0.815669690204649,-0.124911173756694,
0.702247233627224));
#8937=CARTESIAN_POINT('Ctrl Pts',(-0.807662468433796,-0.0925528133349865,
0.711269279199861));
#8938=CARTESIAN_POINT('Ctrl Pts',(-0.803348093619616,-0.05953,0.716109245731214));
#8939=CARTESIAN_POINT('Origin',(-0.991065754692661,-0.05953,0.477272113029314));
#8940=CARTESIAN_POINT('Origin',(0.,-0.05953,0.));
#8941=CARTESIAN_POINT('',(-1.076188,-0.05953,1.31795018948079E-16));
#8942=CARTESIAN_POINT('Origin',(0.,-0.05953,0.));
#8943=CARTESIAN_POINT('',(-1.06075609691358,-0.05953,-0.181596019242328));
#8944=CARTESIAN_POINT('Origin',(0.,-0.05953,0.));
#8945=CARTESIAN_POINT('Origin',(-0.991065754692661,-0.05953,-0.477272113029314));
#8946=CARTESIAN_POINT('Origin',(-0.991065754692661,0.,-0.477272113029314));
#8947=CARTESIAN_POINT('',(-0.803348093619616,-0.05953,-0.716109245731215));
#8948=CARTESIAN_POINT('Ctrl Pts',(-0.803348093619616,-0.05953,-0.716109245731215));
#8949=CARTESIAN_POINT('Ctrl Pts',(-0.807662468433795,-0.0925528133349865,
-0.711269279199862));
#8950=CARTESIAN_POINT('Ctrl Pts',(-0.815669690204649,-0.124911173756694,
-0.702247233627224));
#8951=CARTESIAN_POINT('Ctrl Pts',(-0.835214876415962,-0.177924977804098,
-0.678808213394124));
#8952=CARTESIAN_POINT('Ctrl Pts',(-0.845715984518854,-0.199697230012983,
-0.66581473268113));
#8953=CARTESIAN_POINT('Ctrl Pts',(-0.868789784891799,-0.237895043532788,
-0.635412538795143));
#8954=CARTESIAN_POINT('Ctrl Pts',(-0.8813524085237,-0.254319232363049,-0.617994461173994));
#8955=CARTESIAN_POINT('Ctrl Pts',(-0.906170138993533,-0.28018331644634,
-0.580957796077826));
#8956=CARTESIAN_POINT('Ctrl Pts',(-0.91968254693063,-0.29104845371857,-0.559515758398093));
#8957=CARTESIAN_POINT('Ctrl Pts',(-0.945943877838127,-0.30527573347708,
-0.51387163140139));
#8958=CARTESIAN_POINT('Ctrl Pts',(-0.958671816228589,-0.308638795020976,
-0.489657758261848));
#8959=CARTESIAN_POINT('Ctrl Pts',(-0.980551951791748,-0.308638795020976,
-0.444223188605045));
#8960=CARTESIAN_POINT('Ctrl Pts',(-0.99154738033959,-0.30527573347708,-0.419174982698463));
#8961=CARTESIAN_POINT('Ctrl Pts',(-1.01085972381132,-0.29104845371857,-0.370184399726282));
#8962=CARTESIAN_POINT('Ctrl Pts',(-1.01919893537026,-0.28018331644634,-0.346251081972725));
#8963=CARTESIAN_POINT('Ctrl Pts',(-1.03268176429485,-0.254319232363049,
-0.303755815985685));
#8964=CARTESIAN_POINT('Ctrl Pts',(-1.03846709802406,-0.237895043532788,
-0.283073967563097));
#8965=CARTESIAN_POINT('Ctrl Pts',(-1.04785021111757,-0.199697230012983,
-0.246078686169302));
#8966=CARTESIAN_POINT('Ctrl Pts',(-1.05146158959546,-0.177924977804098,
-0.229767286538461));
#8967=CARTESIAN_POINT('Ctrl Pts',(-1.05760072925372,-0.124911173756694,
-0.199872254546858));
#8968=CARTESIAN_POINT('Ctrl Pts',(-1.05966202740332,-0.0925528133349864,
-0.187986803072857));
#8969=CARTESIAN_POINT('Ctrl Pts',(-1.06075609691358,-0.05953,-0.181596019242328));
#8970=CARTESIAN_POINT('Origin',(-0.991065754692661,-0.05953,-0.477272113029314));
#8971=CARTESIAN_POINT('Origin',(0.,-0.05953,0.));
#8972=CARTESIAN_POINT('',(-0.519393123750572,-0.05953,-0.942555777842682));
#8973=CARTESIAN_POINT('Origin',(0.,-0.05953,0.));
#8974=CARTESIAN_POINT('Origin',(-0.244773027351946,-0.05953,-1.07242070340001));
#8975=CARTESIAN_POINT('Origin',(-0.244773027351946,0.,-1.07242070340001));
#8976=CARTESIAN_POINT('',(0.0589974094846125,-0.05953,-1.07456964270265));
#8977=CARTESIAN_POINT('Ctrl Pts',(0.0589974094846127,-0.05953,-1.07456964270265));
#8978=CARTESIAN_POINT('Ctrl Pts',(0.0525234025782722,-0.0925528133349865,
-1.07492508698591));
#8979=CARTESIAN_POINT('Ctrl Pts',(0.0404772621979744,-0.124911173756694,
-1.07556023164702));
#8980=CARTESIAN_POINT('Ctrl Pts',(0.0099656739833481,-0.177924977804098,
-1.07622728347683));
#8981=CARTESIAN_POINT('Ctrl Pts',(-0.00674037211528096,-0.199697230012983,
-1.07633607767727));
#8982=CARTESIAN_POINT('Ctrl Pts',(-0.044896043654098,-0.237895043532788,
-1.07542044338697));
#8983=CARTESIAN_POINT('Ctrl Pts',(-0.0663467128214644,-0.254319232363049,
-1.07438230428002));
#8984=CARTESIAN_POINT('Ctrl Pts',(-0.110776745452493,-0.28018331644634,
-1.07069360430242));
#8985=CARTESIAN_POINT('Ctrl Pts',(-0.135965654106109,-0.29104845371857,
-1.06788913840721));
#8986=CARTESIAN_POINT('Ctrl Pts',(-0.188025341585962,-0.30527573347708,
-1.05996242598502));
#8987=CARTESIAN_POINT('Ctrl Pts',(-0.214892249704082,-0.308638795020976,
-1.05481642595959));
#8988=CARTESIAN_POINT('Ctrl Pts',(-0.264056468041074,-0.308638795020976,
-1.04359501395068));
#8989=CARTESIAN_POINT('Ctrl Pts',(-0.290495481564827,-0.30527573347708,
-1.036574285215));
#8990=CARTESIAN_POINT('Ctrl Pts',(-0.340838910881557,-0.291048453718569,
-1.02112815447116));
#8991=CARTESIAN_POINT('Ctrl Pts',(-0.364750145543744,-0.28018331644634,
-1.01272583306292));
#8992=CARTESIAN_POINT('Ctrl Pts',(-0.406380688682952,-0.254319232363049,
-0.996771768218699));
#8993=CARTESIAN_POINT('Ctrl Pts',(-0.426157505475872,-0.237895043532788,
-0.988400002689705));
#8994=CARTESIAN_POINT('Ctrl Pts',(-0.460931856495794,-0.199697230012983,
-0.972669835243841));
#8995=CARTESIAN_POINT('Ctrl Pts',(-0.475936279901919,-0.177924977804098,
-0.965323333309091));
#8996=CARTESIAN_POINT('Ctrl Pts',(-0.503136848051454,-0.124911173756694,
-0.951483858396181));
#8997=CARTESIAN_POINT('Ctrl Pts',(-0.513714466572041,-0.0925528133349865,
-0.945684988399766));
#8998=CARTESIAN_POINT('Ctrl Pts',(-0.519393123750572,-0.05953,-0.942555777842682));
#8999=CARTESIAN_POINT('Origin',(-0.244773027351946,-0.05953,-1.07242070340001));
#9000=CARTESIAN_POINT('Origin',(0.,-0.05953,0.));
#9001=CARTESIAN_POINT('',(0.413083465285518,-0.05953,-0.993751811093549));
#9002=CARTESIAN_POINT('Origin',(0.,-0.05953,0.));
#9003=CARTESIAN_POINT('Origin',(0.685838782044607,-0.05953,-0.860014630714833));
#9004=CARTESIAN_POINT('Origin',(0.685838782044607,0.,-0.860014630714833));
#9005=CARTESIAN_POINT('',(0.876916659919095,-0.05953,-0.623857181492959));
#9006=CARTESIAN_POINT('Ctrl Pts',(0.876916659919095,-0.05953,-0.623857181492958));
#9007=CARTESIAN_POINT('Ctrl Pts',(0.873158080166742,-0.0925528133349865,
-0.62914037979579));
#9008=CARTESIAN_POINT('Ctrl Pts',(0.866144010579847,-0.124911173756694,
-0.638954437806245));
#9009=CARTESIAN_POINT('Ctrl Pts',(0.847641868610495,-0.177924977804098,
-0.663225258065736));
#9010=CARTESIAN_POINT('Ctrl Pts',(0.837310877969633,-0.199697230012983,
-0.676354402927683));
#9011=CARTESIAN_POINT('Ctrl Pts',(0.81280533416753,-0.237895043532788,-0.705614819529209));
#9012=CARTESIAN_POINT('Ctrl Pts',(0.798619410861634,-0.254319232363049,
-0.721738358858166));
#9013=CARTESIAN_POINT('Ctrl Pts',(0.768033796848072,-0.28018331644634,-0.754175290318038));
#9014=CARTESIAN_POINT('Ctrl Pts',(0.750136149454208,-0.29104845371857,-0.772120216227122));
#9015=CARTESIAN_POINT('Ctrl Pts',(0.711480111898423,-0.30527573347708,-0.807879894508811));
#9016=CARTESIAN_POINT('Ctrl Pts',(0.690705563850638,-0.308638795020976,
-0.825676810575913));
#9017=CARTESIAN_POINT('Ctrl Pts',(0.651278921914856,-0.308638795020976,
-0.857118508332695));
#9018=CARTESIAN_POINT('Ctrl Pts',(0.629305439856167,-0.30527573347708,-0.873412008702649));
#9019=CARTESIAN_POINT('Ctrl Pts',(0.585840553788742,-0.29104845371857,-0.903141581680914));
#9020=CARTESIAN_POINT('Ctrl Pts',(0.564362943424239,-0.28018331644634,-0.916597376014514));
#9021=CARTESIAN_POINT('Ctrl Pts',(0.525933334162556,-0.254319232363049,
-0.939198248544427));
#9022=CARTESIAN_POINT('Ctrl Pts',(0.507057380724533,-0.237895043532788,
-0.949440676105255));
#9023=CARTESIAN_POINT('Ctrl Pts',(0.473077587363686,-0.199697230012983,
-0.966820759530997));
#9024=CARTESIAN_POINT('Ctrl Pts',(0.457978755888596,-0.177924977804098,
-0.973971221090534));
#9025=CARTESIAN_POINT('Ctrl Pts',(0.430199341854858,-0.124911173756694,
-0.986608710139579));
#9026=CARTESIAN_POINT('Ctrl Pts',(0.419070565453384,-0.0925528133349865,
-0.991263089003441));
#9027=CARTESIAN_POINT('Ctrl Pts',(0.413083465285518,-0.05953,-0.993751811093549));
#9028=CARTESIAN_POINT('Origin',(0.685838782044607,-0.05953,-0.860014630714833));
#9029=CARTESIAN_POINT('Origin',(0.,-0.208355,0.));
#9030=CARTESIAN_POINT('',(-1.076188,-0.35718,1.31795018948079E-16));
#9031=CARTESIAN_POINT('Origin',(0.,-0.35718,0.));
#9032=CARTESIAN_POINT('',(-1.076188,-0.208355,1.31795018948079E-16));
#9033=CARTESIAN_POINT('',(1.03449977959455,-0.05953,0.296632461748266));
#9034=CARTESIAN_POINT('Origin',(0.,-0.05953,0.));
#9035=CARTESIAN_POINT('',(1.03449977959455,-0.05953,-0.296632461748266));
#9036=CARTESIAN_POINT('Ctrl Pts',(1.03449977959455,-0.05953,0.296632461748267));
#9037=CARTESIAN_POINT('Ctrl Pts',(1.03628691421076,-0.0925528133349865,
0.290399865505497));
#9038=CARTESIAN_POINT('Ctrl Pts',(1.03958665287714,-0.124911173756694,0.278797079997872));
#9039=CARTESIAN_POINT('Ctrl Pts',(1.0470264474309,-0.177924977804098,0.249198913998601));
#9040=CARTESIAN_POINT('Ctrl Pts',(1.05084995891418,-0.199697230012983,0.232935932341942));
#9041=CARTESIAN_POINT('Ctrl Pts',(1.05844771715377,-0.237895043532788,0.195533155353269));
#9042=CARTESIAN_POINT('Ctrl Pts',(1.06220882929878,-0.254319232363049,0.17438929156337));
#9043=CARTESIAN_POINT('Ctrl Pts',(1.06849922508772,-0.28018331644634,0.130252399648131));
#9044=CARTESIAN_POINT('Ctrl Pts',(1.07137013248666,-0.29104845371857,0.105070977154072));
#9045=CARTESIAN_POINT('Ctrl Pts',(1.07522652957392,-0.30527573347708,0.0525526752791107));
#9046=CARTESIAN_POINT('Ctrl Pts',(1.076188,-0.308638795020976,0.025214283908933));
#9047=CARTESIAN_POINT('Ctrl Pts',(1.076188,-0.308638795020976,-0.025214283908933));
#9048=CARTESIAN_POINT('Ctrl Pts',(1.07522652957392,-0.30527573347708,-0.0525526752791107));
#9049=CARTESIAN_POINT('Ctrl Pts',(1.07137013248666,-0.29104845371857,-0.105070977154072));
#9050=CARTESIAN_POINT('Ctrl Pts',(1.06849922508772,-0.28018331644634,-0.130252399648131));
#9051=CARTESIAN_POINT('Ctrl Pts',(1.06220882929878,-0.254319232363049,-0.17438929156337));
#9052=CARTESIAN_POINT('Ctrl Pts',(1.05844771715377,-0.237895043532788,-0.195533155353269));
#9053=CARTESIAN_POINT('Ctrl Pts',(1.05084995891418,-0.199697230012983,-0.232935932341942));
#9054=CARTESIAN_POINT('Ctrl Pts',(1.0470264474309,-0.177924977804098,-0.249198913998601));
#9055=CARTESIAN_POINT('Ctrl Pts',(1.03958665287714,-0.124911173756694,-0.278797079997872));
#9056=CARTESIAN_POINT('Ctrl Pts',(1.03628691421076,-0.0925528133349865,
-0.290399865505497));
#9057=CARTESIAN_POINT('Ctrl Pts',(1.03449977959455,-0.05953,-0.296632461748267));
#9058=CARTESIAN_POINT('Origin',(0.,-0.05953,0.));
#9059=CARTESIAN_POINT('Origin',(0.,-0.05953,0.));
#9060=CARTESIAN_POINT('Origin',(1.1,-0.05953,0.));
#9061=CARTESIAN_POINT('Origin',(1.1,0.,0.));
#9062=CARTESIAN_POINT('Origin',(1.1,-0.05953,0.));
#9063=CARTESIAN_POINT('Origin',(0.,-0.35718,0.));
#9064=CARTESIAN_POINT('Origin',(0.,-0.05953,0.));
#10448=UNCERTAINTY_MEASURE_WITH_UNIT(LENGTH_MEASURE(0.001),#10511,
'DISTANCE_ACCURACY_VALUE',
'Maximum model space distance between geometric entities at asserted c
onnectivities');
#10471=UNCERTAINTY_MEASURE_WITH_UNIT(LENGTH_MEASURE(0.001),#10511,
'DISTANCE_ACCURACY_VALUE',
'Maximum model space distance between geometric entities at asserted c
onnectivities');
#10487=(
GEOMETRIC_REPRESENTATION_CONTEXT(3)
GLOBAL_UNCERTAINTY_ASSIGNED_CONTEXT((#10448))
GLOBAL_UNIT_ASSIGNED_CONTEXT((#10511,#10513,#10514))
REPRESENTATION_CONTEXT('','3D')
);
#10510=(
GEOMETRIC_REPRESENTATION_CONTEXT(3)
GLOBAL_UNCERTAINTY_ASSIGNED_CONTEXT((#10471))
GLOBAL_UNIT_ASSIGNED_CONTEXT((#10511,#10513,#10514))
REPRESENTATION_CONTEXT('','3D')
);
#10511=(
LENGTH_UNIT()
NAMED_UNIT(*)
SI_UNIT(.CENTI.,.METRE.)
);
#10513=(
NAMED_UNIT(*)
PLANE_ANGLE_UNIT()
SI_UNIT($,.RADIAN.)
);
#10514=(
NAMED_UNIT(*)
SI_UNIT($,.STERADIAN.)
SOLID_ANGLE_UNIT()
);
#10530=SHAPE_DEFINITION_REPRESENTATION(#10568,#10660);
#10568=PRODUCT_DEFINITION_SHAPE('',$,#10699);
#10660=SHAPE_REPRESENTATION('',(#5918),#10487);
#10683=PRODUCT_DEFINITION_CONTEXT('part definition',#10799,'design');
#10699=PRODUCT_DEFINITION('Cage','Cage',#10737,#10683);
#10737=PRODUCT_DEFINITION_FORMATION('',$,#10816);
#10799=APPLICATION_CONTEXT(
'Core Data for Automotive Mechanical Design Process');
#10800=PRODUCT_CONTEXT('part definition',#10799,'mechanical');
#10816=PRODUCT('Cage','Cage','Cage',(#10800));
#10902=COLOUR_RGB('Grey',0.48,0.52,0.57);
#10903=FILL_AREA_STYLE_COLOUR('',#10902);
#10904=FILL_AREA_STYLE('',(#10903));
#10905=SURFACE_STYLE_FILL_AREA(#10904);
#10906=SURFACE_SIDE_STYLE('',(#10905));
#10907=SURFACE_STYLE_USAGE(.BOTH.,#10906);
#10908=PRESENTATION_STYLE_ASSIGNMENT((#10907));
ENDSEC;
END-ISO-10303-21;
